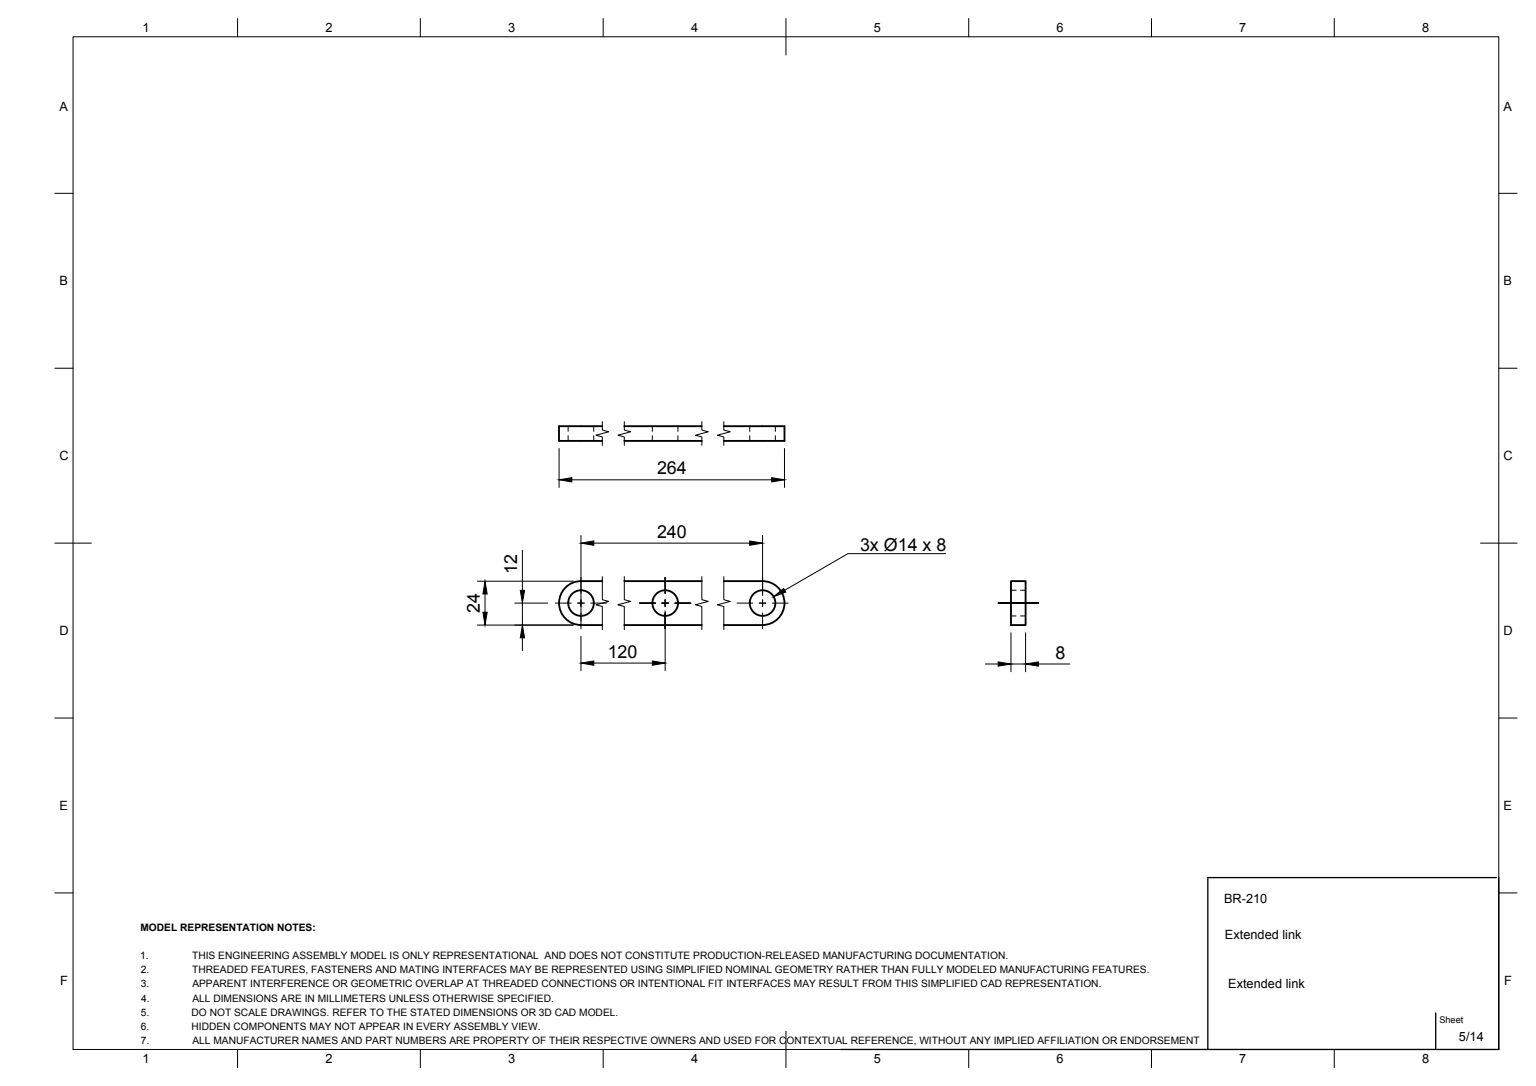
ISO-10303-21;
HEADER;
/* Generated by software containing ST-Developer
 * from STEP Tools, Inc. (www.steptools.com) 
 */

FILE_DESCRIPTION(
/* description */ ('Independent 1:2 reduction pantograph. 120 mm parallelogram sides; fix
ed fulcrum on the extension of a 240 mm link. Drawing point halfway al
ong its link, so its XY displacement is one half of the tracing point.
 Replaceable pivot bushes and retained pins. Calibration and productio
n accuracy unassigned.'),
/* implementation_level */ '2;1');

FILE_NAME(
/* name */ 'Extended link.step',
/* time_stamp */ '2026-11-07T22:11:57-08:00',
/* author */ (''),
/* organization */ (''),
/* preprocessor_version */ 'ST-DEVELOPER v20.2',
/* originating_system */ 'Autodesk Translation Framework v15.17.0.0',
/* authorisation */ '');

FILE_SCHEMA (('AUTOMOTIVE_DESIGN { 1 0 10303 214 3 1 1 }'));
ENDSEC;

DATA;
#10=MECHANICAL_DESIGN_GEOMETRIC_PRESENTATION_REPRESENTATION('',(#188),#2926);
#162=SHAPE_REPRESENTATION_RELATIONSHIP('SRR','None',#2999,#175);
#175=ADVANCED_BREP_SHAPE_REPRESENTATION('',(#201),#2915);
#188=STYLED_ITEM('',(#3073),#201);
#201=MANIFOLD_SOLID_BREP('Body1',#1543);
#224=FACE_BOUND('',#432,.T.);
#225=FACE_BOUND('',#433,.T.);
#226=FACE_BOUND('',#434,.T.);
#227=FACE_BOUND('',#436,.T.);
#228=FACE_BOUND('',#437,.T.);
#229=FACE_BOUND('',#438,.T.);
#266=PLANE('',#1740);
#267=PLANE('',#1744);
#268=PLANE('',#1748);
#269=PLANE('',#1749);
#320=FACE_OUTER_BOUND('',#424,.T.);
#321=FACE_OUTER_BOUND('',#425,.T.);
#322=FACE_OUTER_BOUND('',#426,.T.);
#323=FACE_OUTER_BOUND('',#427,.T.);
#324=FACE_OUTER_BOUND('',#428,.T.);
#325=FACE_OUTER_BOUND('',#429,.T.);
#326=FACE_OUTER_BOUND('',#430,.T.);
#327=FACE_OUTER_BOUND('',#431,.T.);
#328=FACE_OUTER_BOUND('',#435,.T.);
#424=EDGE_LOOP('',(#1133,#1134,#1135,#1136));
#425=EDGE_LOOP('',(#1137,#1138,#1139,#1140));
#426=EDGE_LOOP('',(#1141,#1142,#1143,#1144));
#427=EDGE_LOOP('',(#1145,#1146,#1147,#1148));
#428=EDGE_LOOP('',(#1149,#1150,#1151,#1152));
#429=EDGE_LOOP('',(#1153,#1154,#1155,#1156));
#430=EDGE_LOOP('',(#1157,#1158,#1159,#1160));
#431=EDGE_LOOP('',(#1161,#1162,#1163,#1164));
#432=EDGE_LOOP('',(#1165));
#433=EDGE_LOOP('',(#1166));
#434=EDGE_LOOP('',(#1167));
#435=EDGE_LOOP('',(#1168,#1169,#1170,#1171));
#436=EDGE_LOOP('',(#1172));
#437=EDGE_LOOP('',(#1173));
#438=EDGE_LOOP('',(#1174));
#554=LINE('',#2550,#635);
#555=LINE('',#2556,#636);
#556=LINE('',#2562,#637);
#557=LINE('',#2567,#638);
#558=LINE('',#2569,#639);
#559=LINE('',#2571,#640);
#560=LINE('',#2572,#641);
#561=LINE('',#2578,#642);
#562=LINE('',#2581,#643);
#563=LINE('',#2583,#644);
#564=LINE('',#2584,#645);
#635=VECTOR('',#2018,7.);
#636=VECTOR('',#2025,7.);
#637=VECTOR('',#2032,7.);
#638=VECTOR('',#2037,10.);
#639=VECTOR('',#2038,10.);
#640=VECTOR('',#2039,10.);
#641=VECTOR('',#2040,10.);
#642=VECTOR('',#2047,10.);
#643=VECTOR('',#2050,10.);
#644=VECTOR('',#2051,10.);
#645=VECTOR('',#2052,10.);
#711=CIRCLE('',#1732,7.);
#712=CIRCLE('',#1733,7.);
#713=CIRCLE('',#1735,7.);
#714=CIRCLE('',#1736,7.);
#715=CIRCLE('',#1738,7.);
#716=CIRCLE('',#1739,7.);
#717=CIRCLE('',#1742,12.);
#718=CIRCLE('',#1743,12.);
#719=CIRCLE('',#1746,12.);
#720=CIRCLE('',#1747,12.);
#807=VERTEX_POINT('',#2547);
#808=VERTEX_POINT('',#2549);
#809=VERTEX_POINT('',#2553);
#810=VERTEX_POINT('',#2555);
#811=VERTEX_POINT('',#2559);
#812=VERTEX_POINT('',#2561);
#813=VERTEX_POINT('',#2565);
#814=VERTEX_POINT('',#2566);
#815=VERTEX_POINT('',#2568);
#816=VERTEX_POINT('',#2570);
#817=VERTEX_POINT('',#2574);
#818=VERTEX_POINT('',#2576);
#819=VERTEX_POINT('',#2580);
#820=VERTEX_POINT('',#2582);
#931=EDGE_CURVE('',#807,#807,#711,.T.);
#932=EDGE_CURVE('',#807,#808,#554,.T.);
#933=EDGE_CURVE('',#808,#808,#712,.T.);
#934=EDGE_CURVE('',#809,#809,#713,.T.);
#935=EDGE_CURVE('',#809,#810,#555,.T.);
#936=EDGE_CURVE('',#810,#810,#714,.T.);
#937=EDGE_CURVE('',#811,#811,#715,.T.);
#938=EDGE_CURVE('',#811,#812,#556,.T.);
#939=EDGE_CURVE('',#812,#812,#716,.T.);
#940=EDGE_CURVE('',#813,#814,#557,.T.);
#941=EDGE_CURVE('',#814,#815,#558,.T.);
#942=EDGE_CURVE('',#816,#815,#559,.T.);
#943=EDGE_CURVE('',#813,#816,#560,.T.);
#944=EDGE_CURVE('',#817,#813,#717,.T.);
#945=EDGE_CURVE('',#818,#816,#718,.T.);
#946=EDGE_CURVE('',#817,#818,#561,.T.);
#947=EDGE_CURVE('',#819,#817,#562,.T.);
#948=EDGE_CURVE('',#820,#818,#563,.T.);
#949=EDGE_CURVE('',#819,#820,#564,.T.);
#950=EDGE_CURVE('',#814,#819,#719,.T.);
#951=EDGE_CURVE('',#815,#820,#720,.T.);
#1133=ORIENTED_EDGE('',*,*,#931,.F.);
#1134=ORIENTED_EDGE('',*,*,#932,.T.);
#1135=ORIENTED_EDGE('',*,*,#933,.F.);
#1136=ORIENTED_EDGE('',*,*,#932,.F.);
#1137=ORIENTED_EDGE('',*,*,#934,.F.);
#1138=ORIENTED_EDGE('',*,*,#935,.T.);
#1139=ORIENTED_EDGE('',*,*,#936,.F.);
#1140=ORIENTED_EDGE('',*,*,#935,.F.);
#1141=ORIENTED_EDGE('',*,*,#937,.F.);
#1142=ORIENTED_EDGE('',*,*,#938,.T.);
#1143=ORIENTED_EDGE('',*,*,#939,.F.);
#1144=ORIENTED_EDGE('',*,*,#938,.F.);
#1145=ORIENTED_EDGE('',*,*,#940,.T.);
#1146=ORIENTED_EDGE('',*,*,#941,.T.);
#1147=ORIENTED_EDGE('',*,*,#942,.F.);
#1148=ORIENTED_EDGE('',*,*,#943,.F.);
#1149=ORIENTED_EDGE('',*,*,#944,.T.);
#1150=ORIENTED_EDGE('',*,*,#943,.T.);
#1151=ORIENTED_EDGE('',*,*,#945,.F.);
#1152=ORIENTED_EDGE('',*,*,#946,.F.);
#1153=ORIENTED_EDGE('',*,*,#947,.T.);
#1154=ORIENTED_EDGE('',*,*,#946,.T.);
#1155=ORIENTED_EDGE('',*,*,#948,.F.);
#1156=ORIENTED_EDGE('',*,*,#949,.F.);
#1157=ORIENTED_EDGE('',*,*,#950,.T.);
#1158=ORIENTED_EDGE('',*,*,#949,.T.);
#1159=ORIENTED_EDGE('',*,*,#951,.F.);
#1160=ORIENTED_EDGE('',*,*,#941,.F.);
#1161=ORIENTED_EDGE('',*,*,#951,.T.);
#1162=ORIENTED_EDGE('',*,*,#948,.T.);
#1163=ORIENTED_EDGE('',*,*,#945,.T.);
#1164=ORIENTED_EDGE('',*,*,#942,.T.);
#1165=ORIENTED_EDGE('',*,*,#931,.T.);
#1166=ORIENTED_EDGE('',*,*,#934,.T.);
#1167=ORIENTED_EDGE('',*,*,#937,.T.);
#1168=ORIENTED_EDGE('',*,*,#950,.F.);
#1169=ORIENTED_EDGE('',*,*,#940,.F.);
#1170=ORIENTED_EDGE('',*,*,#944,.F.);
#1171=ORIENTED_EDGE('',*,*,#947,.F.);
#1172=ORIENTED_EDGE('',*,*,#933,.T.);
#1173=ORIENTED_EDGE('',*,*,#936,.T.);
#1174=ORIENTED_EDGE('',*,*,#939,.T.);
#1412=CYLINDRICAL_SURFACE('',#1731,7.);
#1413=CYLINDRICAL_SURFACE('',#1734,7.);
#1414=CYLINDRICAL_SURFACE('',#1737,7.);
#1415=CYLINDRICAL_SURFACE('',#1741,12.);
#1416=CYLINDRICAL_SURFACE('',#1745,12.);
#1464=ADVANCED_FACE('',(#320),#1412,.F.);
#1465=ADVANCED_FACE('',(#321),#1413,.F.);
#1466=ADVANCED_FACE('',(#322),#1414,.F.);
#1467=ADVANCED_FACE('',(#323),#266,.T.);
#1468=ADVANCED_FACE('',(#324),#1415,.T.);
#1469=ADVANCED_FACE('',(#325),#267,.T.);
#1470=ADVANCED_FACE('',(#326),#1416,.T.);
#1471=ADVANCED_FACE('',(#327,#224,#225,#226),#268,.T.);
#1472=ADVANCED_FACE('',(#328,#227,#228,#229),#269,.F.);
#1543=CLOSED_SHELL('',(#1464,#1465,#1466,#1467,#1468,#1469,#1470,#1471,
#1472));
#1730=AXIS2_PLACEMENT_3D('',#2545,#2012,#2013);
#1731=AXIS2_PLACEMENT_3D('',#2546,#2014,#2015);
#1732=AXIS2_PLACEMENT_3D('',#2548,#2016,#2017);
#1733=AXIS2_PLACEMENT_3D('',#2551,#2019,#2020);
#1734=AXIS2_PLACEMENT_3D('',#2552,#2021,#2022);
#1735=AXIS2_PLACEMENT_3D('',#2554,#2023,#2024);
#1736=AXIS2_PLACEMENT_3D('',#2557,#2026,#2027);
#1737=AXIS2_PLACEMENT_3D('',#2558,#2028,#2029);
#1738=AXIS2_PLACEMENT_3D('',#2560,#2030,#2031);
#1739=AXIS2_PLACEMENT_3D('',#2563,#2033,#2034);
#1740=AXIS2_PLACEMENT_3D('',#2564,#2035,#2036);
#1741=AXIS2_PLACEMENT_3D('',#2573,#2041,#2042);
#1742=AXIS2_PLACEMENT_3D('',#2575,#2043,#2044);
#1743=AXIS2_PLACEMENT_3D('',#2577,#2045,#2046);
#1744=AXIS2_PLACEMENT_3D('',#2579,#2048,#2049);
#1745=AXIS2_PLACEMENT_3D('',#2585,#2053,#2054);
#1746=AXIS2_PLACEMENT_3D('',#2586,#2055,#2056);
#1747=AXIS2_PLACEMENT_3D('',#2587,#2057,#2058);
#1748=AXIS2_PLACEMENT_3D('',#2588,#2059,#2060);
#1749=AXIS2_PLACEMENT_3D('',#2589,#2061,#2062);
#2012=DIRECTION('axis',(0.,0.,1.));
#2013=DIRECTION('refdir',(1.,0.,0.));
#2014=DIRECTION('center_axis',(0.,0.,-1.));
#2015=DIRECTION('ref_axis',(1.,0.,0.));
#2016=DIRECTION('center_axis',(0.,0.,-1.));
#2017=DIRECTION('ref_axis',(1.,0.,0.));
#2018=DIRECTION('',(0.,0.,-1.));
#2019=DIRECTION('center_axis',(0.,0.,1.));
#2020=DIRECTION('ref_axis',(1.,0.,0.));
#2021=DIRECTION('center_axis',(0.,0.,-1.));
#2022=DIRECTION('ref_axis',(1.,0.,0.));
#2023=DIRECTION('center_axis',(0.,0.,-1.));
#2024=DIRECTION('ref_axis',(1.,0.,0.));
#2025=DIRECTION('',(0.,0.,-1.));
#2026=DIRECTION('center_axis',(0.,0.,1.));
#2027=DIRECTION('ref_axis',(1.,0.,0.));
#2028=DIRECTION('center_axis',(0.,0.,-1.));
#2029=DIRECTION('ref_axis',(1.,0.,0.));
#2030=DIRECTION('center_axis',(0.,0.,-1.));
#2031=DIRECTION('ref_axis',(1.,0.,0.));
#2032=DIRECTION('',(0.,0.,-1.));
#2033=DIRECTION('center_axis',(0.,0.,1.));
#2034=DIRECTION('ref_axis',(1.,0.,0.));
#2035=DIRECTION('center_axis',(0.,1.,0.));
#2036=DIRECTION('ref_axis',(-1.,0.,0.));
#2037=DIRECTION('',(-1.,0.,0.));
#2038=DIRECTION('',(0.,0.,1.));
#2039=DIRECTION('',(-1.,0.,0.));
#2040=DIRECTION('',(0.,0.,1.));
#2041=DIRECTION('center_axis',(0.,0.,1.));
#2042=DIRECTION('ref_axis',(0.,-1.,0.));
#2043=DIRECTION('center_axis',(0.,0.,1.));
#2044=DIRECTION('ref_axis',(0.,-1.,0.));
#2045=DIRECTION('center_axis',(0.,0.,1.));
#2046=DIRECTION('ref_axis',(0.,-1.,0.));
#2047=DIRECTION('',(0.,0.,1.));
#2048=DIRECTION('center_axis',(0.,-1.,0.));
#2049=DIRECTION('ref_axis',(1.,0.,0.));
#2050=DIRECTION('',(1.,0.,0.));
#2051=DIRECTION('',(1.,0.,0.));
#2052=DIRECTION('',(0.,0.,1.));
#2053=DIRECTION('center_axis',(0.,0.,1.));
#2054=DIRECTION('ref_axis',(0.,1.,0.));
#2055=DIRECTION('center_axis',(0.,0.,1.));
#2056=DIRECTION('ref_axis',(0.,1.,0.));
#2057=DIRECTION('center_axis',(0.,0.,1.));
#2058=DIRECTION('ref_axis',(0.,1.,0.));
#2059=DIRECTION('center_axis',(0.,0.,1.));
#2060=DIRECTION('ref_axis',(1.,0.,0.));
#2061=DIRECTION('center_axis',(0.,0.,1.));
#2062=DIRECTION('ref_axis',(1.,0.,0.));
#2545=CARTESIAN_POINT('',(0.,0.,0.));
#2546=CARTESIAN_POINT('Origin',(120.,0.,4.));
#2547=CARTESIAN_POINT('',(113.,8.57252759403147E-16,8.));
#2548=CARTESIAN_POINT('Origin',(120.,0.,8.));
#2549=CARTESIAN_POINT('',(113.,8.57252759403147E-16,0.));
#2550=CARTESIAN_POINT('',(113.,8.57252759403147E-16,4.));
#2551=CARTESIAN_POINT('Origin',(120.,0.,0.));
#2552=CARTESIAN_POINT('Origin',(0.,0.,4.));
#2553=CARTESIAN_POINT('',(-7.,8.57252759403147E-16,8.));
#2554=CARTESIAN_POINT('Origin',(0.,0.,8.));
#2555=CARTESIAN_POINT('',(-7.,8.57252759403147E-16,0.));
#2556=CARTESIAN_POINT('',(-7.,8.57252759403147E-16,4.));
#2557=CARTESIAN_POINT('Origin',(0.,0.,0.));
#2558=CARTESIAN_POINT('Origin',(240.,0.,4.));
#2559=CARTESIAN_POINT('',(233.,8.57252759403147E-16,8.));
#2560=CARTESIAN_POINT('Origin',(240.,0.,8.));
#2561=CARTESIAN_POINT('',(233.,8.57252759403147E-16,0.));
#2562=CARTESIAN_POINT('',(233.,8.57252759403147E-16,4.));
#2563=CARTESIAN_POINT('Origin',(240.,0.,0.));
#2564=CARTESIAN_POINT('Origin',(240.,12.,0.));
#2565=CARTESIAN_POINT('',(240.,12.,0.));
#2566=CARTESIAN_POINT('',(0.,12.,0.));
#2567=CARTESIAN_POINT('',(240.,12.,0.));
#2568=CARTESIAN_POINT('',(0.,12.,8.));
#2569=CARTESIAN_POINT('',(0.,12.,0.));
#2570=CARTESIAN_POINT('',(240.,12.,8.));
#2571=CARTESIAN_POINT('',(240.,12.,8.));
#2572=CARTESIAN_POINT('',(240.,12.,0.));
#2573=CARTESIAN_POINT('Origin',(240.,-1.11022302462516E-15,0.));
#2574=CARTESIAN_POINT('',(240.,-12.,0.));
#2575=CARTESIAN_POINT('Origin',(240.,-1.11022302462516E-15,0.));
#2576=CARTESIAN_POINT('',(240.,-12.,8.));
#2577=CARTESIAN_POINT('Origin',(240.,-1.11022302462516E-15,8.));
#2578=CARTESIAN_POINT('',(240.,-12.,0.));
#2579=CARTESIAN_POINT('Origin',(0.,-12.,0.));
#2580=CARTESIAN_POINT('',(-1.46957615897682E-15,-12.,0.));
#2581=CARTESIAN_POINT('',(0.,-12.,0.));
#2582=CARTESIAN_POINT('',(-1.46957615897682E-15,-12.,8.));
#2583=CARTESIAN_POINT('',(0.,-12.,8.));
#2584=CARTESIAN_POINT('',(-1.46957615897682E-15,-12.,0.));
#2585=CARTESIAN_POINT('Origin',(0.,0.,0.));
#2586=CARTESIAN_POINT('Origin',(0.,0.,0.));
#2587=CARTESIAN_POINT('Origin',(0.,0.,8.));
#2588=CARTESIAN_POINT('Origin',(120.,0.,8.));
#2589=CARTESIAN_POINT('Origin',(120.,0.,0.));
#2900=UNCERTAINTY_MEASURE_WITH_UNIT(LENGTH_MEASURE(0.01),#2927,
'DISTANCE_ACCURACY_VALUE',
'Maximum model space distance between geometric entities at asserted c
onnectivities');
#2911=UNCERTAINTY_MEASURE_WITH_UNIT(LENGTH_MEASURE(0.01),#2927,
'DISTANCE_ACCURACY_VALUE',
'Maximum model space distance between geometric entities at asserted c
onnectivities');
#2915=(
GEOMETRIC_REPRESENTATION_CONTEXT(3)
GLOBAL_UNCERTAINTY_ASSIGNED_CONTEXT((#2900))
GLOBAL_UNIT_ASSIGNED_CONTEXT((#2927,#2929,#2930))
REPRESENTATION_CONTEXT('','3D')
);
#2926=(
GEOMETRIC_REPRESENTATION_CONTEXT(3)
GLOBAL_UNCERTAINTY_ASSIGNED_CONTEXT((#2911))
GLOBAL_UNIT_ASSIGNED_CONTEXT((#2927,#2929,#2930))
REPRESENTATION_CONTEXT('','3D')
);
#2927=(
LENGTH_UNIT()
NAMED_UNIT(*)
SI_UNIT(.MILLI.,.METRE.)
);
#2929=(
NAMED_UNIT(*)
PLANE_ANGLE_UNIT()
SI_UNIT($,.RADIAN.)
);
#2930=(
NAMED_UNIT(*)
SI_UNIT($,.STERADIAN.)
SOLID_ANGLE_UNIT()
);
#2934=SHAPE_DEFINITION_REPRESENTATION(#2948,#2999);
#2948=PRODUCT_DEFINITION_SHAPE('',$,#3014);
#2999=SHAPE_REPRESENTATION('',(#1730),#2915);
#3010=PRODUCT_DEFINITION_CONTEXT('part definition',#3054,'design');
#3014=PRODUCT_DEFINITION('Extended link','Extended link',#3028,#3010);
#3028=PRODUCT_DEFINITION_FORMATION('',$,#3059);
#3054=APPLICATION_CONTEXT(
'Core Data for Automotive Mechanical Design Process');
#3055=PRODUCT_CONTEXT('part definition',#3054,'mechanical');
#3059=PRODUCT('Extended link','Extended link',$,(#3055));
#3073=PRESENTATION_STYLE_ASSIGNMENT((#3085));
#3085=SURFACE_STYLE_USAGE(.BOTH.,#3097);
#3097=SURFACE_SIDE_STYLE('',(#3109));
#3109=SURFACE_STYLE_FILL_AREA(#3121);
#3121=FILL_AREA_STYLE('Extended link finish',(#3133));
#3133=FILL_AREA_STYLE_COLOUR('Extended link finish',#3145);
#3145=COLOUR_RGB('Extended link finish',0.0901960784313725,0.270588235294118,
0.513725490196078);
ENDSEC;
END-ISO-10303-21;
